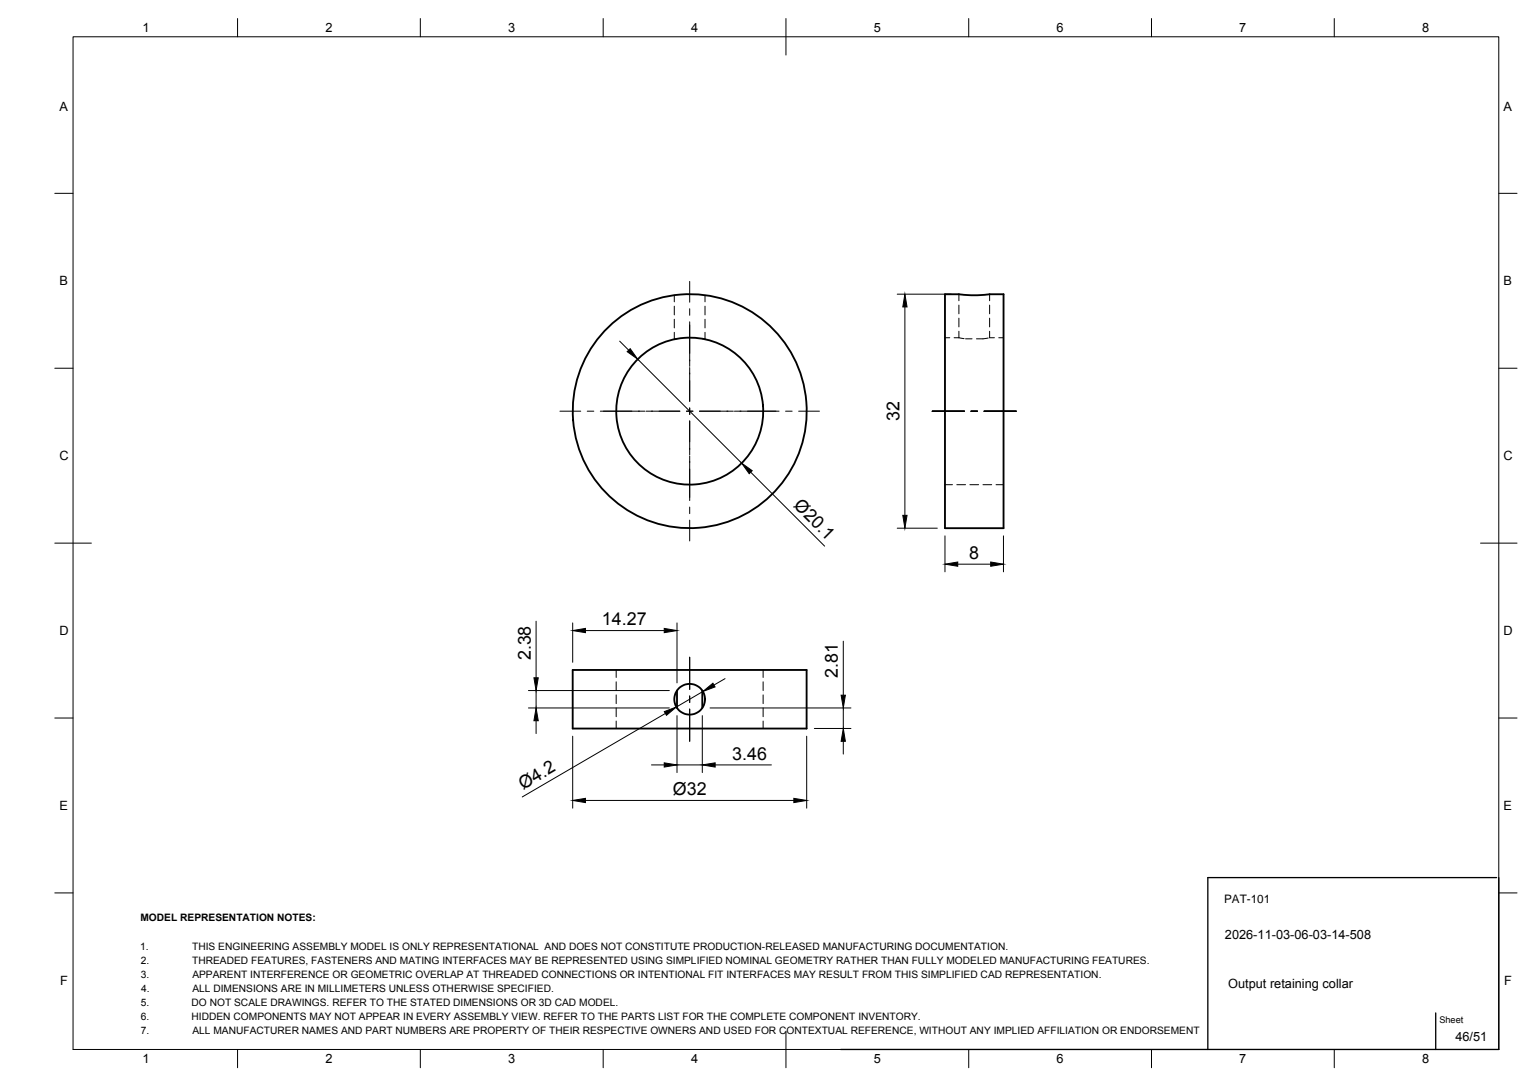
ISO-10303-21;
HEADER;
/* Generated by software containing ST-Developer
 * from STEP Tools, Inc. (www.steptools.com) 
 */

FILE_DESCRIPTION(
/* description */ ('Spur gear reduction stage 2-1 on bearing plates'),
/* implementation_level */ '2;1');

FILE_NAME(
/* name */ 'Output retaining collar.step',
/* time_stamp */ '2026-10-28T03:22:07-07:00',
/* author */ (''),
/* organization */ (''),
/* preprocessor_version */ 'ST-DEVELOPER v20.2',
/* originating_system */ 'Autodesk Translation Framework v15.17.0.0',
/* authorisation */ '');

FILE_SCHEMA (('AUTOMOTIVE_DESIGN { 1 0 10303 214 3 1 1 }'));
ENDSEC;

DATA;
#10=MECHANICAL_DESIGN_GEOMETRIC_PRESENTATION_REPRESENTATION('',(#998),#53909);
#707=B_SPLINE_CURVE_WITH_KNOTS('',3,(#29914,#29915,#29916,#29917,#29918,
#29919,#29920,#29921,#29922,#29923,#29924,#29925,#29926,#29927),
 .UNSPECIFIED.,.F.,.F.,(4,2,2,2,2,2,4),(0.75600573798701,0.793568827564648,
0.872922520054202,0.952276212543757,1.03162990503331,1.11098359752287,1.1485466871005),
 .UNSPECIFIED.);
#708=B_SPLINE_CURVE_WITH_KNOTS('',3,(#29933,#29934,#29935,#29936,#29937,
#29938,#29939,#29940,#29941,#29942,#29943,#29944,#29945,#29946,#29947,#29948,
#29949,#29950),.UNSPECIFIED.,.F.,.F.,(4,2,2,2,2,2,2,2,4),(0.,0.0792028026112442,
0.158405605222488,0.237607602356378,0.316809599490267,0.396011596624156,
0.475213593758045,0.554416396369289,0.633619198980534),.UNSPECIFIED.);
#709=B_SPLINE_CURVE_WITH_KNOTS('',3,(#29951,#29952,#29953,#29954,#29955,
#29956,#29957,#29958,#29959,#29960,#29961,#29962,#29963,#29964,#29965,#29966,
#29967,#29968),.UNSPECIFIED.,.F.,.F.,(4,2,2,2,2,2,2,2,4),(0.633619198980534,
0.712822001591778,0.792024804203022,0.871226801336911,0.9504287984708,1.02963079560469,
1.10883279273858,1.18803559534982,1.26723839796107),.UNSPECIFIED.);
#710=B_SPLINE_CURVE_WITH_KNOTS('',3,(#29971,#29972,#29973,#29974,#29975,
#29976,#29977,#29978,#29979,#29980,#29981,#29982,#29983,#29984),
 .UNSPECIFIED.,.F.,.F.,(4,2,2,2,2,2,4),(0.121154929624505,0.158718019202143,
0.238071711691698,0.317425404181252,0.396779096670807,0.476132789160362,
0.513695878738),.UNSPECIFIED.);
#897=SHAPE_REPRESENTATION_RELATIONSHIP('SRR','None',#54128,#940);
#940=ADVANCED_BREP_SHAPE_REPRESENTATION('',(#1053),#53902);
#998=STYLED_ITEM('',(#54411),#1053);
#1053=MANIFOLD_SOLID_BREP('Body1',#11325);
#1222=FACE_BOUND('',#2753,.T.);
#1223=FACE_BOUND('',#2755,.T.);
#1224=FACE_BOUND('',#2757,.T.);
#1225=FACE_BOUND('',#2759,.T.);
#1426=PLANE('',#12709);
#1427=PLANE('',#12714);
#1428=PLANE('',#12721);
#1429=PLANE('',#12722);
#1939=FACE_OUTER_BOUND('',#2749,.T.);
#1940=FACE_OUTER_BOUND('',#2750,.T.);
#1941=FACE_OUTER_BOUND('',#2751,.T.);
#1942=FACE_OUTER_BOUND('',#2752,.T.);
#1943=FACE_OUTER_BOUND('',#2754,.T.);
#1944=FACE_OUTER_BOUND('',#2756,.T.);
#1945=FACE_OUTER_BOUND('',#2758,.T.);
#2749=EDGE_LOOP('',(#9244,#9245));
#2750=EDGE_LOOP('',(#9246,#9247,#9248,#9249,#9250,#9251,#9252,#9253,#9254));
#2751=EDGE_LOOP('',(#9255,#9256,#9257));
#2752=EDGE_LOOP('',(#9258,#9259,#9260,#9261));
#2753=EDGE_LOOP('',(#9262,#9263,#9264,#9265));
#2754=EDGE_LOOP('',(#9266,#9267,#9268,#9269));
#2755=EDGE_LOOP('',(#9270,#9271));
#2756=EDGE_LOOP('',(#9272));
#2757=EDGE_LOOP('',(#9273));
#2758=EDGE_LOOP('',(#9274));
#2759=EDGE_LOOP('',(#9275));
#3388=LINE('',#29910,#4029);
#3389=LINE('',#29931,#4030);
#3390=LINE('',#29986,#4031);
#3391=LINE('',#29991,#4032);
#3392=LINE('',#29997,#4033);
#4029=VECTOR('',#15201,1.);
#4030=VECTOR('',#15208,0.21);
#4031=VECTOR('',#15213,1.);
#4032=VECTOR('',#15218,1.005);
#4033=VECTOR('',#15225,1.6);
#4674=CIRCLE('',#12710,0.21);
#4675=CIRCLE('',#12712,0.21);
#4676=CIRCLE('',#12713,0.21);
#4677=CIRCLE('',#12716,1.005);
#4678=CIRCLE('',#12717,1.005);
#4679=CIRCLE('',#12719,1.6);
#4680=CIRCLE('',#12720,1.6);
#5426=VERTEX_POINT('',#29908);
#5427=VERTEX_POINT('',#29909);
#5428=VERTEX_POINT('',#29913);
#5429=VERTEX_POINT('',#29928);
#5430=VERTEX_POINT('',#29930);
#5431=VERTEX_POINT('',#29932);
#5432=VERTEX_POINT('',#29969);
#5433=VERTEX_POINT('',#29988);
#5434=VERTEX_POINT('',#29990);
#5435=VERTEX_POINT('',#29994);
#5436=VERTEX_POINT('',#29996);
#6764=EDGE_CURVE('',#5426,#5427,#3388,.T.);
#6765=EDGE_CURVE('',#5426,#5427,#4674,.T.);
#6766=EDGE_CURVE('',#5428,#5426,#707,.T.);
#6767=EDGE_CURVE('',#5429,#5428,#4675,.T.);
#6768=EDGE_CURVE('',#5429,#5430,#3389,.T.);
#6769=EDGE_CURVE('',#5431,#5430,#708,.T.);
#6770=EDGE_CURVE('',#5430,#5431,#709,.T.);
#6771=EDGE_CURVE('',#5432,#5429,#4676,.T.);
#6772=EDGE_CURVE('',#5427,#5432,#710,.T.);
#6773=EDGE_CURVE('',#5432,#5428,#3390,.T.);
#6774=EDGE_CURVE('',#5433,#5433,#4677,.T.);
#6775=EDGE_CURVE('',#5433,#5434,#3391,.T.);
#6776=EDGE_CURVE('',#5434,#5434,#4678,.T.);
#6777=EDGE_CURVE('',#5435,#5435,#4679,.T.);
#6778=EDGE_CURVE('',#5435,#5436,#3392,.T.);
#6779=EDGE_CURVE('',#5436,#5436,#4680,.T.);
#9244=ORIENTED_EDGE('',*,*,#6764,.F.);
#9245=ORIENTED_EDGE('',*,*,#6765,.T.);
#9246=ORIENTED_EDGE('',*,*,#6766,.F.);
#9247=ORIENTED_EDGE('',*,*,#6767,.F.);
#9248=ORIENTED_EDGE('',*,*,#6768,.T.);
#9249=ORIENTED_EDGE('',*,*,#6769,.F.);
#9250=ORIENTED_EDGE('',*,*,#6770,.F.);
#9251=ORIENTED_EDGE('',*,*,#6768,.F.);
#9252=ORIENTED_EDGE('',*,*,#6771,.F.);
#9253=ORIENTED_EDGE('',*,*,#6772,.F.);
#9254=ORIENTED_EDGE('',*,*,#6765,.F.);
#9255=ORIENTED_EDGE('',*,*,#6773,.F.);
#9256=ORIENTED_EDGE('',*,*,#6771,.T.);
#9257=ORIENTED_EDGE('',*,*,#6767,.T.);
#9258=ORIENTED_EDGE('',*,*,#6774,.F.);
#9259=ORIENTED_EDGE('',*,*,#6775,.T.);
#9260=ORIENTED_EDGE('',*,*,#6776,.T.);
#9261=ORIENTED_EDGE('',*,*,#6775,.F.);
#9262=ORIENTED_EDGE('',*,*,#6772,.T.);
#9263=ORIENTED_EDGE('',*,*,#6773,.T.);
#9264=ORIENTED_EDGE('',*,*,#6766,.T.);
#9265=ORIENTED_EDGE('',*,*,#6764,.T.);
#9266=ORIENTED_EDGE('',*,*,#6777,.F.);
#9267=ORIENTED_EDGE('',*,*,#6778,.T.);
#9268=ORIENTED_EDGE('',*,*,#6779,.T.);
#9269=ORIENTED_EDGE('',*,*,#6778,.F.);
#9270=ORIENTED_EDGE('',*,*,#6769,.T.);
#9271=ORIENTED_EDGE('',*,*,#6770,.T.);
#9272=ORIENTED_EDGE('',*,*,#6777,.T.);
#9273=ORIENTED_EDGE('',*,*,#6774,.T.);
#9274=ORIENTED_EDGE('',*,*,#6779,.F.);
#9275=ORIENTED_EDGE('',*,*,#6776,.F.);
#10570=CYLINDRICAL_SURFACE('',#12711,0.21);
#10571=CYLINDRICAL_SURFACE('',#12715,1.005);
#10572=CYLINDRICAL_SURFACE('',#12718,1.6);
#11059=ADVANCED_FACE('',(#1939),#1426,.T.);
#11060=ADVANCED_FACE('',(#1940),#10570,.F.);
#11061=ADVANCED_FACE('',(#1941),#1427,.T.);
#11062=ADVANCED_FACE('',(#1942,#1222),#10571,.F.);
#11063=ADVANCED_FACE('',(#1943,#1223),#10572,.T.);
#11064=ADVANCED_FACE('',(#1944,#1224),#1428,.T.);
#11065=ADVANCED_FACE('',(#1945,#1225),#1429,.F.);
#11325=CLOSED_SHELL('',(#11059,#11060,#11061,#11062,#11063,#11064,#11065));
#12708=AXIS2_PLACEMENT_3D('',#29906,#15197,#15198);
#12709=AXIS2_PLACEMENT_3D('',#29907,#15199,#15200);
#12710=AXIS2_PLACEMENT_3D('',#29911,#15202,#15203);
#12711=AXIS2_PLACEMENT_3D('',#29912,#15204,#15205);
#12712=AXIS2_PLACEMENT_3D('',#29929,#15206,#15207);
#12713=AXIS2_PLACEMENT_3D('',#29970,#15209,#15210);
#12714=AXIS2_PLACEMENT_3D('',#29985,#15211,#15212);
#12715=AXIS2_PLACEMENT_3D('',#29987,#15214,#15215);
#12716=AXIS2_PLACEMENT_3D('',#29989,#15216,#15217);
#12717=AXIS2_PLACEMENT_3D('',#29992,#15219,#15220);
#12718=AXIS2_PLACEMENT_3D('',#29993,#15221,#15222);
#12719=AXIS2_PLACEMENT_3D('',#29995,#15223,#15224);
#12720=AXIS2_PLACEMENT_3D('',#29998,#15226,#15227);
#12721=AXIS2_PLACEMENT_3D('',#29999,#15228,#15229);
#12722=AXIS2_PLACEMENT_3D('',#30000,#15230,#15231);
#15197=DIRECTION('axis',(0.,0.,1.));
#15198=DIRECTION('refdir',(1.,0.,0.));
#15199=DIRECTION('center_axis',(0.,0.,1.));
#15200=DIRECTION('ref_axis',(1.,0.,0.));
#15201=DIRECTION('',(0.,1.,0.));
#15202=DIRECTION('center_axis',(0.,0.,1.));
#15203=DIRECTION('ref_axis',(1.,0.,0.));
#15204=DIRECTION('center_axis',(0.,0.,1.));
#15205=DIRECTION('ref_axis',(1.,0.,0.));
#15206=DIRECTION('center_axis',(0.,0.,1.));
#15207=DIRECTION('ref_axis',(1.,0.,0.));
#15208=DIRECTION('',(0.,0.,1.));
#15209=DIRECTION('center_axis',(0.,0.,1.));
#15210=DIRECTION('ref_axis',(1.,0.,0.));
#15211=DIRECTION('center_axis',(0.,0.,1.));
#15212=DIRECTION('ref_axis',(1.,0.,0.));
#15213=DIRECTION('',(0.,-1.,0.));
#15214=DIRECTION('center_axis',(0.,1.,0.));
#15215=DIRECTION('ref_axis',(1.,0.,0.));
#15216=DIRECTION('center_axis',(0.,-1.,0.));
#15217=DIRECTION('ref_axis',(1.,0.,0.));
#15218=DIRECTION('',(0.,-1.,0.));
#15219=DIRECTION('center_axis',(0.,-1.,0.));
#15220=DIRECTION('ref_axis',(1.,0.,0.));
#15221=DIRECTION('center_axis',(0.,1.,0.));
#15222=DIRECTION('ref_axis',(1.,0.,0.));
#15223=DIRECTION('center_axis',(0.,1.,0.));
#15224=DIRECTION('ref_axis',(1.,0.,0.));
#15225=DIRECTION('',(0.,-1.,0.));
#15226=DIRECTION('center_axis',(0.,1.,0.));
#15227=DIRECTION('ref_axis',(1.,0.,0.));
#15228=DIRECTION('center_axis',(0.,1.,0.));
#15229=DIRECTION('ref_axis',(1.,0.,0.));
#15230=DIRECTION('center_axis',(0.,1.,0.));
#15231=DIRECTION('ref_axis',(1.,0.,0.));
#29906=CARTESIAN_POINT('',(0.,0.,0.));
#29907=CARTESIAN_POINT('Origin',(0.,-5.1,0.99));
#29908=CARTESIAN_POINT('',(0.172988438920062,-5.21905880899791,0.99));
#29909=CARTESIAN_POINT('',(0.172988438920062,-4.98094119100209,0.99));
#29910=CARTESIAN_POINT('',(0.172988438920062,-5.5,0.99));
#29911=CARTESIAN_POINT('Origin',(0.,-5.1,0.99));
#29912=CARTESIAN_POINT('Origin',(0.,-5.1,0.99));
#29913=CARTESIAN_POINT('',(-0.172988438920062,-5.21905880899791,0.99));
#29914=CARTESIAN_POINT('Ctrl Pts',(-0.172988438920062,-5.21905880899791,
0.99));
#29915=CARTESIAN_POINT('Ctrl Pts',(-0.165594865311319,-5.22980142239529,
0.991291921976381));
#29916=CARTESIAN_POINT('Ctrl Pts',(-0.157297138725609,-5.23968770937274,
0.992653949439047));
#29917=CARTESIAN_POINT('Ctrl Pts',(-0.129892073845076,-5.26709277425327,
0.996748084390898));
#29918=CARTESIAN_POINT('Ctrl Pts',(-0.106330167759284,-5.28324205633295,
0.999695893276376));
#29919=CARTESIAN_POINT('Ctrl Pts',(-0.05461290463241,-5.30469779396491,
1.00385029472357));
#29920=CARTESIAN_POINT('Ctrl Pts',(-0.0264512308298516,-5.31,1.005));
#29921=CARTESIAN_POINT('Ctrl Pts',(0.0264512308298516,-5.31,1.005));
#29922=CARTESIAN_POINT('Ctrl Pts',(0.054612904632411,-5.30469779396491,
1.00385029472357));
#29923=CARTESIAN_POINT('Ctrl Pts',(0.106330167759285,-5.28324205633295,
0.999695893276376));
#29924=CARTESIAN_POINT('Ctrl Pts',(0.129892073845076,-5.26709277425327,
0.996748084390898));
#29925=CARTESIAN_POINT('Ctrl Pts',(0.157297138725609,-5.23968770937274,
0.992653949439047));
#29926=CARTESIAN_POINT('Ctrl Pts',(0.165594865311319,-5.22980142239529,
0.991291921976381));
#29927=CARTESIAN_POINT('Ctrl Pts',(0.172988438920062,-5.21905880899791,
0.99));
#29928=CARTESIAN_POINT('',(-0.21,-5.1,0.99));
#29929=CARTESIAN_POINT('Origin',(0.,-5.1,0.99));
#29930=CARTESIAN_POINT('',(-0.21,-5.1,1.58615888233178));
#29931=CARTESIAN_POINT('',(-0.21,-5.1,0.99));
#29932=CARTESIAN_POINT('',(0.21,-5.1,1.58615888233178));
#29933=CARTESIAN_POINT('Ctrl Pts',(0.21,-5.1,1.58615888233178));
#29934=CARTESIAN_POINT('Ctrl Pts',(0.21,-5.12640093420375,1.58615888233178));
#29935=CARTESIAN_POINT('Ctrl Pts',(0.20471752266132,-5.15454055536511,1.58688606295397));
#29936=CARTESIAN_POINT('Ctrl Pts',(0.183276841782292,-5.2062710523005,1.58950502964782));
#29937=CARTESIAN_POINT('Ctrl Pts',(0.167120287247804,-5.22986456085055,
1.59135816887013));
#29938=CARTESIAN_POINT('Ctrl Pts',(0.129864750292352,-5.267120097806,1.59483075953278));
#29939=CARTESIAN_POINT('Ctrl Pts',(0.106271159541076,-5.28327680083123,
1.59667690933009));
#29940=CARTESIAN_POINT('Ctrl Pts',(0.0545403836274689,-5.3047175903444,
1.59927985626981));
#29941=CARTESIAN_POINT('Ctrl Pts',(0.0264006657112964,-5.31,1.6));
#29942=CARTESIAN_POINT('Ctrl Pts',(-0.0264006657112964,-5.31,1.6));
#29943=CARTESIAN_POINT('Ctrl Pts',(-0.0545403836274682,-5.3047175903444,
1.59927985626981));
#29944=CARTESIAN_POINT('Ctrl Pts',(-0.106271159541075,-5.28327680083123,
1.59667690933009));
#29945=CARTESIAN_POINT('Ctrl Pts',(-0.129864750292352,-5.267120097806,1.59483075953278));
#29946=CARTESIAN_POINT('Ctrl Pts',(-0.167120287247804,-5.22986456085055,
1.59135816887013));
#29947=CARTESIAN_POINT('Ctrl Pts',(-0.183276841782292,-5.2062710523005,
1.58950502964782));
#29948=CARTESIAN_POINT('Ctrl Pts',(-0.20471752266132,-5.15454055536511,
1.58688606295397));
#29949=CARTESIAN_POINT('Ctrl Pts',(-0.21,-5.12640093420375,1.58615888233178));
#29950=CARTESIAN_POINT('Ctrl Pts',(-0.21,-5.1,1.58615888233178));
#29951=CARTESIAN_POINT('Ctrl Pts',(-0.21,-5.1,1.58615888233178));
#29952=CARTESIAN_POINT('Ctrl Pts',(-0.21,-5.07359906579625,1.58615888233178));
#29953=CARTESIAN_POINT('Ctrl Pts',(-0.20471752266132,-5.04545944463489,
1.58688606295397));
#29954=CARTESIAN_POINT('Ctrl Pts',(-0.183276841782292,-4.9937289476995,
1.58950502964782));
#29955=CARTESIAN_POINT('Ctrl Pts',(-0.167120287247804,-4.97013543914945,
1.59135816887013));
#29956=CARTESIAN_POINT('Ctrl Pts',(-0.129864750292352,-4.932879902194,1.59483075953278));
#29957=CARTESIAN_POINT('Ctrl Pts',(-0.106271159541076,-4.91672319916876,
1.59667690933009));
#29958=CARTESIAN_POINT('Ctrl Pts',(-0.0545403836274689,-4.8952824096556,
1.59927985626981));
#29959=CARTESIAN_POINT('Ctrl Pts',(-0.0264006657112965,-4.89,1.6));
#29960=CARTESIAN_POINT('Ctrl Pts',(0.0264006657112964,-4.89,1.6));
#29961=CARTESIAN_POINT('Ctrl Pts',(0.0545403836274682,-4.8952824096556,
1.59927985626981));
#29962=CARTESIAN_POINT('Ctrl Pts',(0.106271159541075,-4.91672319916876,
1.59667690933009));
#29963=CARTESIAN_POINT('Ctrl Pts',(0.129864750292352,-4.932879902194,1.59483075953278));
#29964=CARTESIAN_POINT('Ctrl Pts',(0.167120287247804,-4.97013543914945,
1.59135816887013));
#29965=CARTESIAN_POINT('Ctrl Pts',(0.183276841782292,-4.9937289476995,1.58950502964782));
#29966=CARTESIAN_POINT('Ctrl Pts',(0.20471752266132,-5.04545944463489,1.58688606295397));
#29967=CARTESIAN_POINT('Ctrl Pts',(0.21,-5.07359906579625,1.58615888233178));
#29968=CARTESIAN_POINT('Ctrl Pts',(0.21,-5.1,1.58615888233178));
#29969=CARTESIAN_POINT('',(-0.172988438920062,-4.98094119100209,0.99));
#29970=CARTESIAN_POINT('Origin',(0.,-5.1,0.99));
#29971=CARTESIAN_POINT('Ctrl Pts',(0.172988438920062,-4.98094119100209,
0.99));
#29972=CARTESIAN_POINT('Ctrl Pts',(0.165594865311318,-4.97019857760471,
0.991291921976381));
#29973=CARTESIAN_POINT('Ctrl Pts',(0.157297138725609,-4.96031229062726,
0.992653949439047));
#29974=CARTESIAN_POINT('Ctrl Pts',(0.129892073845076,-4.93290722574673,
0.996748084390898));
#29975=CARTESIAN_POINT('Ctrl Pts',(0.106330167759284,-4.91675794366705,
0.999695893276376));
#29976=CARTESIAN_POINT('Ctrl Pts',(0.05461290463241,-4.89530220603509,1.00385029472357));
#29977=CARTESIAN_POINT('Ctrl Pts',(0.0264512308298516,-4.89,1.005));
#29978=CARTESIAN_POINT('Ctrl Pts',(-0.0264512308298516,-4.89,1.005));
#29979=CARTESIAN_POINT('Ctrl Pts',(-0.05461290463241,-4.89530220603509,
1.00385029472357));
#29980=CARTESIAN_POINT('Ctrl Pts',(-0.106330167759284,-4.91675794366705,
0.999695893276376));
#29981=CARTESIAN_POINT('Ctrl Pts',(-0.129892073845076,-4.93290722574673,
0.996748084390898));
#29982=CARTESIAN_POINT('Ctrl Pts',(-0.157297138725609,-4.96031229062726,
0.992653949439047));
#29983=CARTESIAN_POINT('Ctrl Pts',(-0.165594865311318,-4.97019857760471,
0.991291921976381));
#29984=CARTESIAN_POINT('Ctrl Pts',(-0.172988438920062,-4.98094119100209,
0.99));
#29985=CARTESIAN_POINT('Origin',(0.,-5.1,0.99));
#29986=CARTESIAN_POINT('',(-0.172988438920062,-5.5,0.99));
#29987=CARTESIAN_POINT('Origin',(0.,-5.5,0.));
#29988=CARTESIAN_POINT('',(-1.005,-4.7,1.23077003314309E-16));
#29989=CARTESIAN_POINT('Origin',(0.,-4.7,0.));
#29990=CARTESIAN_POINT('',(-1.005,-5.5,1.23077003314309E-16));
#29991=CARTESIAN_POINT('',(-1.005,-5.5,1.23077003314309E-16));
#29992=CARTESIAN_POINT('Origin',(0.,-5.5,0.));
#29993=CARTESIAN_POINT('Origin',(0.,-5.5,0.));
#29994=CARTESIAN_POINT('',(-1.6,-4.7,1.95943487863577E-16));
#29995=CARTESIAN_POINT('Origin',(0.,-4.7,0.));
#29996=CARTESIAN_POINT('',(-1.6,-5.5,1.95943487863577E-16));
#29997=CARTESIAN_POINT('',(-1.6,-5.5,1.95943487863577E-16));
#29998=CARTESIAN_POINT('Origin',(0.,-5.5,0.));
#29999=CARTESIAN_POINT('Origin',(0.,-4.7,0.));
#30000=CARTESIAN_POINT('Origin',(0.,-5.5,0.));
#53852=UNCERTAINTY_MEASURE_WITH_UNIT(LENGTH_MEASURE(0.001),#53910,
'DISTANCE_ACCURACY_VALUE',
'Maximum model space distance between geometric entities at asserted c
onnectivities');
#53859=UNCERTAINTY_MEASURE_WITH_UNIT(LENGTH_MEASURE(0.001),#53910,
'DISTANCE_ACCURACY_VALUE',
'Maximum model space distance between geometric entities at asserted c
onnectivities');
#53902=(
GEOMETRIC_REPRESENTATION_CONTEXT(3)
GLOBAL_UNCERTAINTY_ASSIGNED_CONTEXT((#53852))
GLOBAL_UNIT_ASSIGNED_CONTEXT((#53910,#53912,#53913))
REPRESENTATION_CONTEXT('','3D')
);
#53909=(
GEOMETRIC_REPRESENTATION_CONTEXT(3)
GLOBAL_UNCERTAINTY_ASSIGNED_CONTEXT((#53859))
GLOBAL_UNIT_ASSIGNED_CONTEXT((#53910,#53912,#53913))
REPRESENTATION_CONTEXT('','3D')
);
#53910=(
LENGTH_UNIT()
NAMED_UNIT(*)
SI_UNIT(.CENTI.,.METRE.)
);
#53912=(
NAMED_UNIT(*)
PLANE_ANGLE_UNIT()
SI_UNIT($,.RADIAN.)
);
#53913=(
NAMED_UNIT(*)
SI_UNIT($,.STERADIAN.)
SOLID_ANGLE_UNIT()
);
#53956=SHAPE_DEFINITION_REPRESENTATION(#54054,#54128);
#54054=PRODUCT_DEFINITION_SHAPE('',$,#54178);
#54128=SHAPE_REPRESENTATION('',(#12708),#53902);
#54135=PRODUCT_DEFINITION_CONTEXT('part definition',#54284,'design');
#54178=PRODUCT_DEFINITION('Output retaining collar',
'Output retaining collar',#54227,#54135);
#54227=PRODUCT_DEFINITION_FORMATION('',$,#54328);
#54284=APPLICATION_CONTEXT(
'Core Data for Automotive Mechanical Design Process');
#54285=PRODUCT_CONTEXT('part definition',#54284,'mechanical');
#54328=PRODUCT('Output retaining collar','Output retaining collar',
'Output retaining collar',(#54285));
#54405=COLOUR_RGB('Off White',0.89,0.88,0.83);
#54406=FILL_AREA_STYLE_COLOUR('',#54405);
#54407=FILL_AREA_STYLE('',(#54406));
#54408=SURFACE_STYLE_FILL_AREA(#54407);
#54409=SURFACE_SIDE_STYLE('',(#54408));
#54410=SURFACE_STYLE_USAGE(.BOTH.,#54409);
#54411=PRESENTATION_STYLE_ASSIGNMENT((#54410));
ENDSEC;
END-ISO-10303-21;
